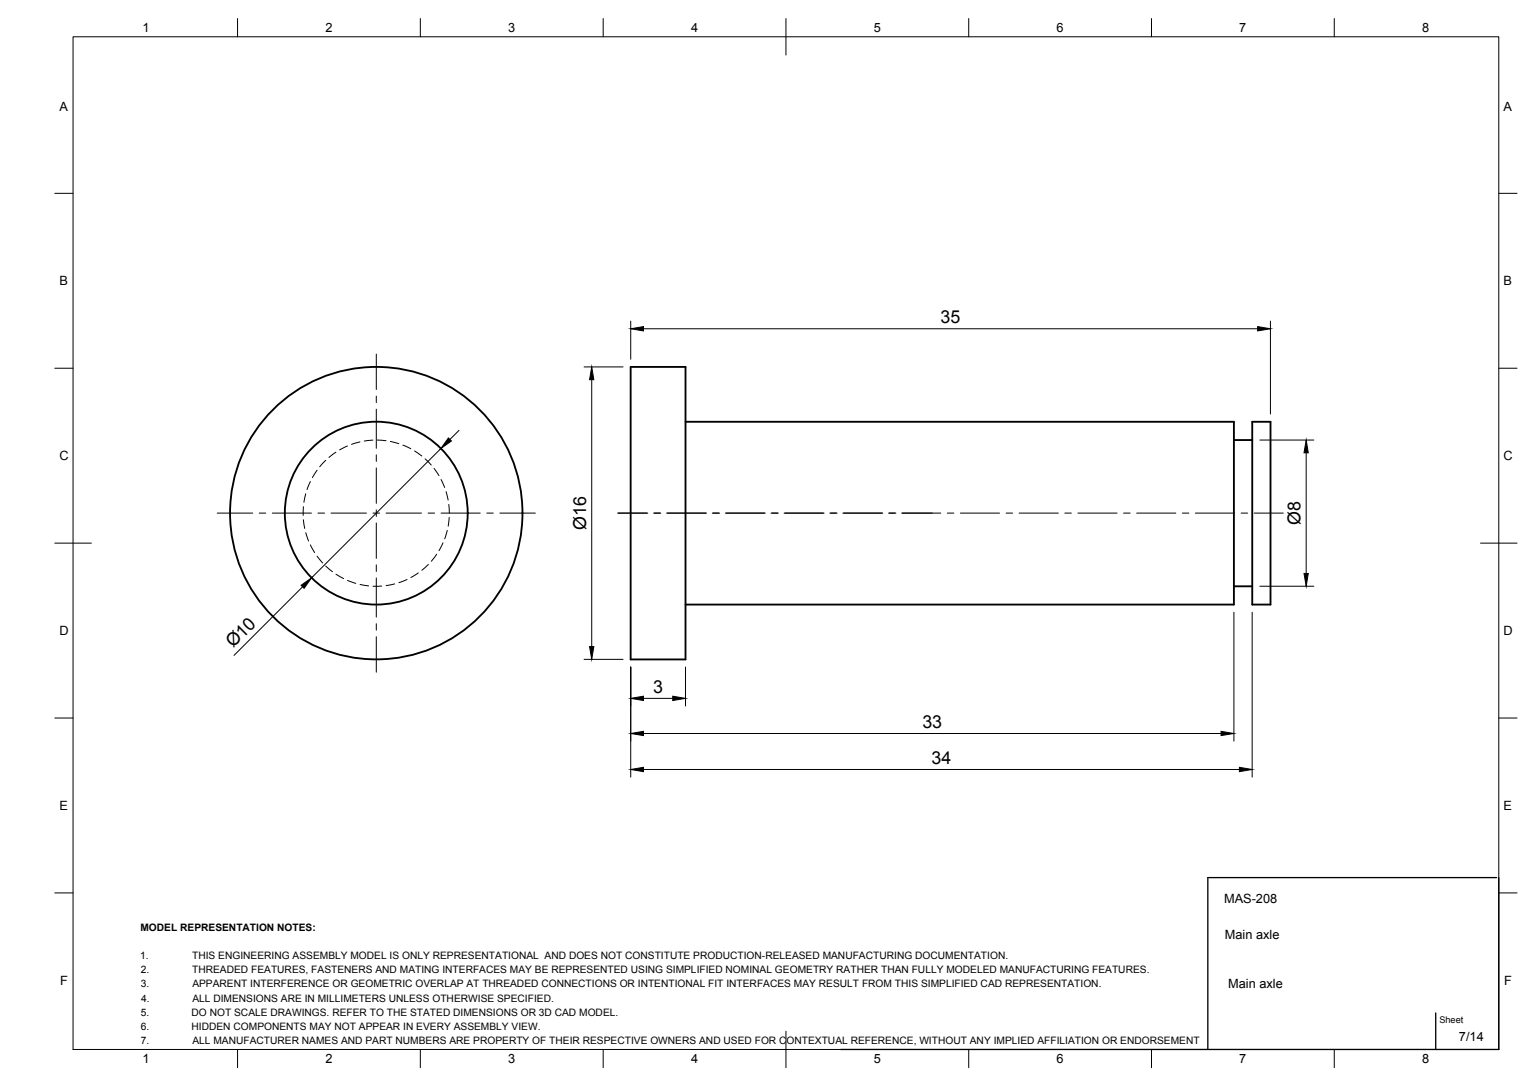
ISO-10303-21;
HEADER;
/* Generated by software containing ST-Developer
 * from STEP Tools, Inc. (www.steptools.com) 
 */

FILE_DESCRIPTION(
/* description */ ('Independent vertical20-tooth ratchet advance with repeated integral-c
ounterweight gravity pawls, swinging drive lever, bronze sleeves and f
ully retained axle stacks.18degpertooth. Native revolutes; geometric c
ycle checking rather than automatic contact/rolling dynamics. Gravity 
closing checked from actual pawl center of mass. Backplate/foot suppor
ts unit. Fits, torque, holding force, wear and life unassigned.'),
/* implementation_level */ '2;1');

FILE_NAME(
/* name */ 'Main axle.step',
/* time_stamp */ '2026-11-09T06:25:53-08:00',
/* author */ (''),
/* organization */ (''),
/* preprocessor_version */ 'ST-DEVELOPER v20.2',
/* originating_system */ 'Autodesk Translation Framework v15.17.0.0',
/* authorisation */ '');

FILE_SCHEMA (('AUTOMOTIVE_DESIGN { 1 0 10303 214 3 1 1 }'));
ENDSEC;

DATA;
#10=MECHANICAL_DESIGN_GEOMETRIC_PRESENTATION_REPRESENTATION('',(#126),#4643);
#98=SHAPE_REPRESENTATION_RELATIONSHIP('SRR','None',#4703,#112);
#112=ADVANCED_BREP_SHAPE_REPRESENTATION('',(#140),#4632);
#126=STYLED_ITEM('',(#4782),#140);
#140=MANIFOLD_SOLID_BREP('Body1',#2662);
#171=FACE_BOUND('',#547,.T.);
#172=FACE_BOUND('',#549,.T.);
#173=FACE_BOUND('',#552,.T.);
#254=PLANE('',#2928);
#255=PLANE('',#2930);
#256=PLANE('',#2934);
#257=PLANE('',#2939);
#258=PLANE('',#2941);
#376=FACE_OUTER_BOUND('',#545,.T.);
#377=FACE_OUTER_BOUND('',#546,.T.);
#378=FACE_OUTER_BOUND('',#548,.T.);
#379=FACE_OUTER_BOUND('',#550,.T.);
#380=FACE_OUTER_BOUND('',#551,.T.);
#381=FACE_OUTER_BOUND('',#553,.T.);
#382=FACE_OUTER_BOUND('',#554,.T.);
#383=FACE_OUTER_BOUND('',#555,.T.);
#384=FACE_OUTER_BOUND('',#556,.T.);
#545=EDGE_LOOP('',(#2197,#2198,#2199,#2200));
#546=EDGE_LOOP('',(#2201));
#547=EDGE_LOOP('',(#2202));
#548=EDGE_LOOP('',(#2203));
#549=EDGE_LOOP('',(#2204));
#550=EDGE_LOOP('',(#2205,#2206,#2207,#2208));
#551=EDGE_LOOP('',(#2209));
#552=EDGE_LOOP('',(#2210));
#553=EDGE_LOOP('',(#2211,#2212,#2213,#2214));
#554=EDGE_LOOP('',(#2215));
#555=EDGE_LOOP('',(#2216,#2217,#2218,#2219));
#556=EDGE_LOOP('',(#2220));
#821=LINE('',#4278,#1083);
#822=LINE('',#4289,#1084);
#823=LINE('',#4297,#1085);
#824=LINE('',#4301,#1086);
#1083=VECTOR('',#3463,4.);
#1084=VECTOR('',#3478,5.);
#1085=VECTOR('',#3487,8.);
#1086=VECTOR('',#3494,5.);
#1187=CIRCLE('',#2926,4.);
#1188=CIRCLE('',#2927,4.);
#1189=CIRCLE('',#2929,5.);
#1190=CIRCLE('',#2931,5.);
#1191=CIRCLE('',#2933,5.);
#1192=CIRCLE('',#2935,8.);
#1193=CIRCLE('',#2936,5.);
#1194=CIRCLE('',#2938,8.);
#1373=VERTEX_POINT('',#4275);
#1374=VERTEX_POINT('',#4277);
#1375=VERTEX_POINT('',#4281);
#1376=VERTEX_POINT('',#4284);
#1377=VERTEX_POINT('',#4287);
#1378=VERTEX_POINT('',#4291);
#1379=VERTEX_POINT('',#4293);
#1380=VERTEX_POINT('',#4296);
#1663=EDGE_CURVE('',#1373,#1373,#1187,.T.);
#1664=EDGE_CURVE('',#1373,#1374,#821,.T.);
#1665=EDGE_CURVE('',#1374,#1374,#1188,.T.);
#1666=EDGE_CURVE('',#1375,#1375,#1189,.T.);
#1667=EDGE_CURVE('',#1376,#1376,#1190,.T.);
#1668=EDGE_CURVE('',#1377,#1377,#1191,.T.);
#1669=EDGE_CURVE('',#1377,#1376,#822,.T.);
#1670=EDGE_CURVE('',#1378,#1378,#1192,.T.);
#1671=EDGE_CURVE('',#1379,#1379,#1193,.T.);
#1672=EDGE_CURVE('',#1378,#1380,#823,.T.);
#1673=EDGE_CURVE('',#1380,#1380,#1194,.T.);
#1674=EDGE_CURVE('',#1375,#1379,#824,.T.);
#2197=ORIENTED_EDGE('',*,*,#1663,.T.);
#2198=ORIENTED_EDGE('',*,*,#1664,.T.);
#2199=ORIENTED_EDGE('',*,*,#1665,.F.);
#2200=ORIENTED_EDGE('',*,*,#1664,.F.);
#2201=ORIENTED_EDGE('',*,*,#1666,.F.);
#2202=ORIENTED_EDGE('',*,*,#1663,.F.);
#2203=ORIENTED_EDGE('',*,*,#1667,.F.);
#2204=ORIENTED_EDGE('',*,*,#1665,.T.);
#2205=ORIENTED_EDGE('',*,*,#1668,.F.);
#2206=ORIENTED_EDGE('',*,*,#1669,.T.);
#2207=ORIENTED_EDGE('',*,*,#1667,.T.);
#2208=ORIENTED_EDGE('',*,*,#1669,.F.);
#2209=ORIENTED_EDGE('',*,*,#1670,.T.);
#2210=ORIENTED_EDGE('',*,*,#1671,.F.);
#2211=ORIENTED_EDGE('',*,*,#1670,.F.);
#2212=ORIENTED_EDGE('',*,*,#1672,.T.);
#2213=ORIENTED_EDGE('',*,*,#1673,.T.);
#2214=ORIENTED_EDGE('',*,*,#1672,.F.);
#2215=ORIENTED_EDGE('',*,*,#1673,.F.);
#2216=ORIENTED_EDGE('',*,*,#1666,.T.);
#2217=ORIENTED_EDGE('',*,*,#1674,.T.);
#2218=ORIENTED_EDGE('',*,*,#1671,.T.);
#2219=ORIENTED_EDGE('',*,*,#1674,.F.);
#2220=ORIENTED_EDGE('',*,*,#1668,.T.);
#2483=CYLINDRICAL_SURFACE('',#2925,4.);
#2484=CYLINDRICAL_SURFACE('',#2932,5.);
#2485=CYLINDRICAL_SURFACE('',#2937,8.);
#2486=CYLINDRICAL_SURFACE('',#2940,5.);
#2582=ADVANCED_FACE('',(#376),#2483,.T.);
#2583=ADVANCED_FACE('',(#377,#171),#254,.F.);
#2584=ADVANCED_FACE('',(#378,#172),#255,.F.);
#2585=ADVANCED_FACE('',(#379),#2484,.T.);
#2586=ADVANCED_FACE('',(#380,#173),#256,.T.);
#2587=ADVANCED_FACE('',(#381),#2485,.T.);
#2588=ADVANCED_FACE('',(#382),#257,.F.);
#2589=ADVANCED_FACE('',(#383),#2486,.T.);
#2590=ADVANCED_FACE('',(#384),#258,.T.);
#2662=CLOSED_SHELL('',(#2582,#2583,#2584,#2585,#2586,#2587,#2588,#2589,
#2590));
#2924=AXIS2_PLACEMENT_3D('',#4273,#3457,#3458);
#2925=AXIS2_PLACEMENT_3D('',#4274,#3459,#3460);
#2926=AXIS2_PLACEMENT_3D('',#4276,#3461,#3462);
#2927=AXIS2_PLACEMENT_3D('',#4279,#3464,#3465);
#2928=AXIS2_PLACEMENT_3D('',#4280,#3466,#3467);
#2929=AXIS2_PLACEMENT_3D('',#4282,#3468,#3469);
#2930=AXIS2_PLACEMENT_3D('',#4283,#3470,#3471);
#2931=AXIS2_PLACEMENT_3D('',#4285,#3472,#3473);
#2932=AXIS2_PLACEMENT_3D('',#4286,#3474,#3475);
#2933=AXIS2_PLACEMENT_3D('',#4288,#3476,#3477);
#2934=AXIS2_PLACEMENT_3D('',#4290,#3479,#3480);
#2935=AXIS2_PLACEMENT_3D('',#4292,#3481,#3482);
#2936=AXIS2_PLACEMENT_3D('',#4294,#3483,#3484);
#2937=AXIS2_PLACEMENT_3D('',#4295,#3485,#3486);
#2938=AXIS2_PLACEMENT_3D('',#4298,#3488,#3489);
#2939=AXIS2_PLACEMENT_3D('',#4299,#3490,#3491);
#2940=AXIS2_PLACEMENT_3D('',#4300,#3492,#3493);
#2941=AXIS2_PLACEMENT_3D('',#4302,#3495,#3496);
#3457=DIRECTION('axis',(0.,0.,1.));
#3458=DIRECTION('refdir',(1.,0.,0.));
#3459=DIRECTION('center_axis',(0.,0.,1.));
#3460=DIRECTION('ref_axis',(1.,0.,0.));
#3461=DIRECTION('center_axis',(0.,0.,1.));
#3462=DIRECTION('ref_axis',(1.,0.,0.));
#3463=DIRECTION('',(0.,0.,1.));
#3464=DIRECTION('center_axis',(0.,0.,1.));
#3465=DIRECTION('ref_axis',(1.,0.,0.));
#3466=DIRECTION('center_axis',(0.,0.,-1.));
#3467=DIRECTION('ref_axis',(-1.,0.,0.));
#3468=DIRECTION('center_axis',(0.,0.,-1.));
#3469=DIRECTION('ref_axis',(1.,0.,0.));
#3470=DIRECTION('center_axis',(0.,0.,1.));
#3471=DIRECTION('ref_axis',(1.,0.,0.));
#3472=DIRECTION('center_axis',(0.,0.,1.));
#3473=DIRECTION('ref_axis',(1.,0.,0.));
#3474=DIRECTION('center_axis',(0.,0.,1.));
#3475=DIRECTION('ref_axis',(1.,0.,0.));
#3476=DIRECTION('center_axis',(0.,0.,1.));
#3477=DIRECTION('ref_axis',(1.,0.,0.));
#3478=DIRECTION('',(0.,0.,-1.));
#3479=DIRECTION('center_axis',(0.,0.,1.));
#3480=DIRECTION('ref_axis',(1.,0.,0.));
#3481=DIRECTION('center_axis',(0.,0.,1.));
#3482=DIRECTION('ref_axis',(1.,0.,0.));
#3483=DIRECTION('center_axis',(0.,0.,1.));
#3484=DIRECTION('ref_axis',(1.,0.,0.));
#3485=DIRECTION('center_axis',(0.,0.,1.));
#3486=DIRECTION('ref_axis',(1.,0.,0.));
#3487=DIRECTION('',(0.,0.,-1.));
#3488=DIRECTION('center_axis',(0.,0.,1.));
#3489=DIRECTION('ref_axis',(1.,0.,0.));
#3490=DIRECTION('center_axis',(0.,0.,1.));
#3491=DIRECTION('ref_axis',(1.,0.,0.));
#3492=DIRECTION('center_axis',(0.,0.,1.));
#3493=DIRECTION('ref_axis',(1.,0.,0.));
#3494=DIRECTION('',(0.,0.,-1.));
#3495=DIRECTION('center_axis',(0.,0.,1.));
#3496=DIRECTION('ref_axis',(1.,0.,0.));
#4273=CARTESIAN_POINT('',(0.,0.,0.));
#4274=CARTESIAN_POINT('Origin',(0.,0.,30.5));
#4275=CARTESIAN_POINT('',(-4.,-4.89858719658941E-16,30.));
#4276=CARTESIAN_POINT('Origin',(0.,0.,30.));
#4277=CARTESIAN_POINT('',(-4.,-4.89858719658941E-16,31.));
#4278=CARTESIAN_POINT('',(-4.,-4.89858719658941E-16,30.5));
#4279=CARTESIAN_POINT('Origin',(0.,0.,31.));
#4280=CARTESIAN_POINT('Origin',(8.,0.,30.));
#4281=CARTESIAN_POINT('',(-5.,6.12323399573677E-16,30.));
#4282=CARTESIAN_POINT('Origin',(0.,0.,30.));
#4283=CARTESIAN_POINT('Origin',(4.,0.,31.));
#4284=CARTESIAN_POINT('',(-5.,-6.12323399573677E-16,31.));
#4285=CARTESIAN_POINT('Origin',(0.,0.,31.));
#4286=CARTESIAN_POINT('Origin',(0.,0.,0.));
#4287=CARTESIAN_POINT('',(-5.,-6.12323399573677E-16,32.));
#4288=CARTESIAN_POINT('Origin',(0.,0.,32.));
#4289=CARTESIAN_POINT('',(-5.,-6.12323399573677E-16,0.));
#4290=CARTESIAN_POINT('Origin',(0.,0.,0.));
#4291=CARTESIAN_POINT('',(-8.,-9.79717439317883E-16,0.));
#4292=CARTESIAN_POINT('Origin',(0.,0.,0.));
#4293=CARTESIAN_POINT('',(-5.,-6.12323399573677E-16,0.));
#4294=CARTESIAN_POINT('Origin',(0.,0.,0.));
#4295=CARTESIAN_POINT('Origin',(0.,0.,-3.));
#4296=CARTESIAN_POINT('',(-8.,-9.79717439317883E-16,-3.));
#4297=CARTESIAN_POINT('',(-8.,-9.79717439317883E-16,-3.));
#4298=CARTESIAN_POINT('Origin',(0.,0.,-3.));
#4299=CARTESIAN_POINT('Origin',(0.,0.,-3.));
#4300=CARTESIAN_POINT('Origin',(0.,0.,0.));
#4301=CARTESIAN_POINT('',(-5.,-6.12323399573677E-16,0.));
#4302=CARTESIAN_POINT('Origin',(0.,0.,32.));
#4616=UNCERTAINTY_MEASURE_WITH_UNIT(LENGTH_MEASURE(0.01),#4644,
'DISTANCE_ACCURACY_VALUE',
'Maximum model space distance between geometric entities at asserted c
onnectivities');
#4627=UNCERTAINTY_MEASURE_WITH_UNIT(LENGTH_MEASURE(0.01),#4644,
'DISTANCE_ACCURACY_VALUE',
'Maximum model space distance between geometric entities at asserted c
onnectivities');
#4632=(
GEOMETRIC_REPRESENTATION_CONTEXT(3)
GLOBAL_UNCERTAINTY_ASSIGNED_CONTEXT((#4616))
GLOBAL_UNIT_ASSIGNED_CONTEXT((#4644,#4646,#4647))
REPRESENTATION_CONTEXT('','3D')
);
#4643=(
GEOMETRIC_REPRESENTATION_CONTEXT(3)
GLOBAL_UNCERTAINTY_ASSIGNED_CONTEXT((#4627))
GLOBAL_UNIT_ASSIGNED_CONTEXT((#4644,#4646,#4647))
REPRESENTATION_CONTEXT('','3D')
);
#4644=(
LENGTH_UNIT()
NAMED_UNIT(*)
SI_UNIT(.MILLI.,.METRE.)
);
#4646=(
NAMED_UNIT(*)
PLANE_ANGLE_UNIT()
SI_UNIT($,.RADIAN.)
);
#4647=(
NAMED_UNIT(*)
SI_UNIT($,.STERADIAN.)
SOLID_ANGLE_UNIT()
);
#4652=SHAPE_DEFINITION_REPRESENTATION(#4667,#4703);
#4667=PRODUCT_DEFINITION_SHAPE('',$,#4719);
#4703=SHAPE_REPRESENTATION('',(#2924),#4632);
#4714=PRODUCT_DEFINITION_CONTEXT('part definition',#4761,'design');
#4719=PRODUCT_DEFINITION('Main axle','Main axle',#4734,#4714);
#4734=PRODUCT_DEFINITION_FORMATION('',$,#4767);
#4761=APPLICATION_CONTEXT(
'Core Data for Automotive Mechanical Design Process');
#4762=PRODUCT_CONTEXT('part definition',#4761,'mechanical');
#4767=PRODUCT('Main axle','Main axle',$,(#4762));
#4782=PRESENTATION_STYLE_ASSIGNMENT((#4791));
#4791=SURFACE_STYLE_USAGE(.BOTH.,#4800);
#4800=SURFACE_SIDE_STYLE('',(#4809));
#4809=SURFACE_STYLE_FILL_AREA(#4818);
#4818=FILL_AREA_STYLE('Axle gray',(#4827));
#4827=FILL_AREA_STYLE_COLOUR('Axle gray',#4836);
#4836=COLOUR_RGB('Axle gray',0.576470588235294,0.615686274509804,0.666666666666667);
ENDSEC;
END-ISO-10303-21;
